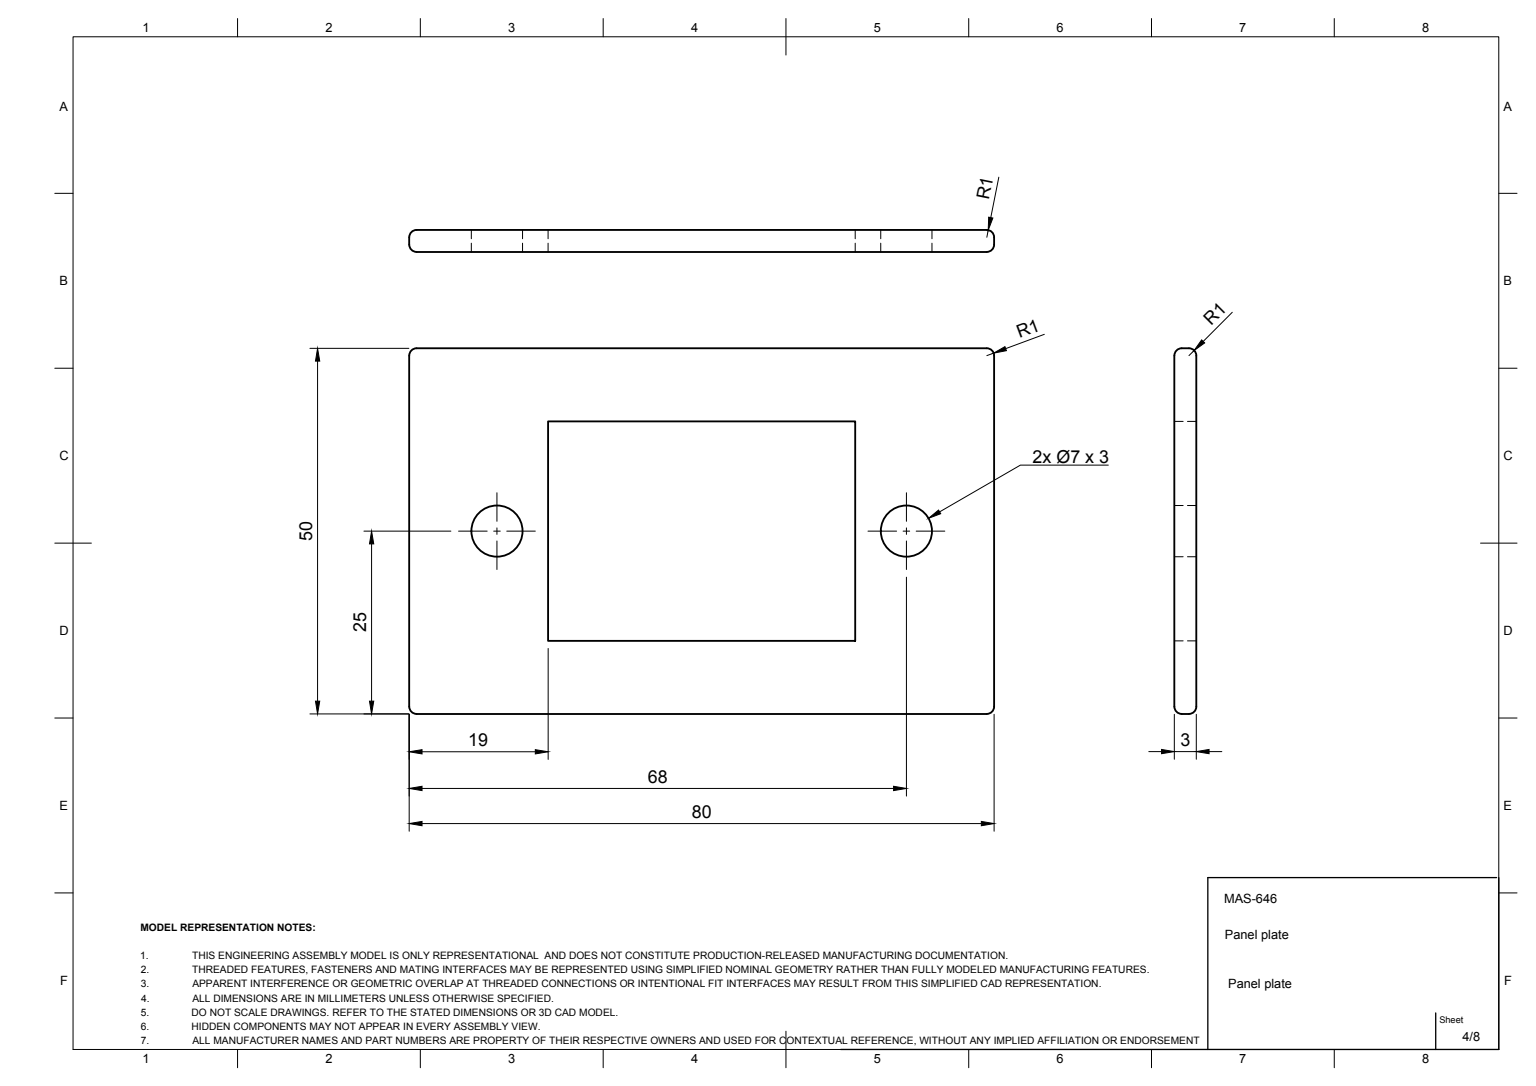
ISO-10303-21;
HEADER;
/* Generated by software containing ST-Developer
 * from STEP Tools, Inc. (www.steptools.com) 
 */

FILE_DESCRIPTION(
/* description */ ('Independent keyed three-contact power inlet for the IEC-connector des
ign category. Longer ground blade, retained contacts, wire termination
 holes and sealed bolted panel interface. Nominal custom interface; IE
C dimensional compatibility and electrical ratings are not assigned.'),

/* implementation_level */ '2;1');

FILE_NAME(
/* name */ 'Panel plate.step',
/* time_stamp */ '2026-11-08T19:55:04-08:00',
/* author */ (''),
/* organization */ (''),
/* preprocessor_version */ 'ST-DEVELOPER v20.2',
/* originating_system */ 'Autodesk Translation Framework v15.17.0.0',
/* authorisation */ '');

FILE_SCHEMA (('AUTOMOTIVE_DESIGN { 1 0 10303 214 3 1 1 }'));
ENDSEC;

DATA;
#10=MECHANICAL_DESIGN_GEOMETRIC_PRESENTATION_REPRESENTATION('',(#110),#21880);
#81=SPHERICAL_SURFACE('',#6694,0.999999999999996);
#82=SPHERICAL_SURFACE('',#6698,0.999999999999996);
#83=SPHERICAL_SURFACE('',#6702,1.);
#84=SPHERICAL_SURFACE('',#6706,0.999999999999996);
#85=SPHERICAL_SURFACE('',#6710,1.);
#86=SPHERICAL_SURFACE('',#6714,0.999999999999996);
#87=SPHERICAL_SURFACE('',#6718,1.);
#88=SPHERICAL_SURFACE('',#6722,1.);
#90=SHAPE_REPRESENTATION_RELATIONSHIP('SRR','None',#21926,#100);
#100=ADVANCED_BREP_SHAPE_REPRESENTATION('',(#120),#21871);
#110=STYLED_ITEM('',(#21985),#120);
#120=MANIFOLD_SOLID_BREP('Body1',#6382);
#159=FACE_BOUND('',#863,.T.);
#160=FACE_BOUND('',#864,.T.);
#161=FACE_BOUND('',#865,.T.);
#162=FACE_BOUND('',#869,.T.);
#163=FACE_BOUND('',#870,.T.);
#164=FACE_BOUND('',#871,.T.);
#233=PLANE('',#6738);
#234=PLANE('',#6739);
#235=PLANE('',#6742);
#236=PLANE('',#6743);
#237=PLANE('',#6744);
#238=PLANE('',#6747);
#239=PLANE('',#6750);
#240=PLANE('',#6751);
#241=PLANE('',#6752);
#242=PLANE('',#6753);
#481=FACE_OUTER_BOUND('',#841,.T.);
#482=FACE_OUTER_BOUND('',#842,.T.);
#483=FACE_OUTER_BOUND('',#843,.T.);
#484=FACE_OUTER_BOUND('',#844,.T.);
#485=FACE_OUTER_BOUND('',#845,.T.);
#486=FACE_OUTER_BOUND('',#846,.T.);
#487=FACE_OUTER_BOUND('',#847,.T.);
#488=FACE_OUTER_BOUND('',#848,.T.);
#489=FACE_OUTER_BOUND('',#849,.T.);
#490=FACE_OUTER_BOUND('',#850,.T.);
#491=FACE_OUTER_BOUND('',#851,.T.);
#492=FACE_OUTER_BOUND('',#852,.T.);
#493=FACE_OUTER_BOUND('',#853,.T.);
#494=FACE_OUTER_BOUND('',#854,.T.);
#495=FACE_OUTER_BOUND('',#855,.T.);
#496=FACE_OUTER_BOUND('',#856,.T.);
#497=FACE_OUTER_BOUND('',#857,.T.);
#498=FACE_OUTER_BOUND('',#858,.T.);
#499=FACE_OUTER_BOUND('',#859,.T.);
#500=FACE_OUTER_BOUND('',#860,.T.);
#501=FACE_OUTER_BOUND('',#861,.T.);
#502=FACE_OUTER_BOUND('',#862,.T.);
#503=FACE_OUTER_BOUND('',#866,.T.);
#504=FACE_OUTER_BOUND('',#867,.T.);
#505=FACE_OUTER_BOUND('',#868,.T.);
#506=FACE_OUTER_BOUND('',#872,.T.);
#507=FACE_OUTER_BOUND('',#873,.T.);
#508=FACE_OUTER_BOUND('',#874,.T.);
#509=FACE_OUTER_BOUND('',#875,.T.);
#510=FACE_OUTER_BOUND('',#876,.T.);
#511=FACE_OUTER_BOUND('',#877,.T.);
#512=FACE_OUTER_BOUND('',#878,.T.);
#841=EDGE_LOOP('',(#4883,#4884,#4885));
#842=EDGE_LOOP('',(#4886,#4887,#4888));
#843=EDGE_LOOP('',(#4889,#4890,#4891));
#844=EDGE_LOOP('',(#4892,#4893,#4894));
#845=EDGE_LOOP('',(#4895,#4896,#4897));
#846=EDGE_LOOP('',(#4898,#4899,#4900));
#847=EDGE_LOOP('',(#4901,#4902,#4903));
#848=EDGE_LOOP('',(#4904,#4905,#4906));
#849=EDGE_LOOP('',(#4907,#4908,#4909,#4910));
#850=EDGE_LOOP('',(#4911,#4912,#4913,#4914));
#851=EDGE_LOOP('',(#4915,#4916,#4917,#4918));
#852=EDGE_LOOP('',(#4919,#4920,#4921,#4922));
#853=EDGE_LOOP('',(#4923,#4924,#4925,#4926));
#854=EDGE_LOOP('',(#4927,#4928,#4929,#4930));
#855=EDGE_LOOP('',(#4931,#4932,#4933,#4934));
#856=EDGE_LOOP('',(#4935,#4936,#4937,#4938));
#857=EDGE_LOOP('',(#4939,#4940,#4941,#4942));
#858=EDGE_LOOP('',(#4943,#4944,#4945,#4946));
#859=EDGE_LOOP('',(#4947,#4948,#4949,#4950));
#860=EDGE_LOOP('',(#4951,#4952,#4953,#4954));
#861=EDGE_LOOP('',(#4955,#4956,#4957,#4958));
#862=EDGE_LOOP('',(#4959,#4960,#4961,#4962));
#863=EDGE_LOOP('',(#4963,#4964,#4965,#4966));
#864=EDGE_LOOP('',(#4967));
#865=EDGE_LOOP('',(#4968));
#866=EDGE_LOOP('',(#4969,#4970,#4971,#4972));
#867=EDGE_LOOP('',(#4973,#4974,#4975,#4976));
#868=EDGE_LOOP('',(#4977,#4978,#4979,#4980));
#869=EDGE_LOOP('',(#4981,#4982,#4983,#4984));
#870=EDGE_LOOP('',(#4985));
#871=EDGE_LOOP('',(#4986));
#872=EDGE_LOOP('',(#4987,#4988,#4989,#4990));
#873=EDGE_LOOP('',(#4991,#4992,#4993,#4994));
#874=EDGE_LOOP('',(#4995,#4996,#4997,#4998));
#875=EDGE_LOOP('',(#4999,#5000,#5001,#5002));
#876=EDGE_LOOP('',(#5003,#5004,#5005,#5006));
#877=EDGE_LOOP('',(#5007,#5008,#5009,#5010));
#878=EDGE_LOOP('',(#5011,#5012,#5013,#5014));
#1096=CIRCLE('',#6695,1.);
#1097=CIRCLE('',#6696,0.999999999999996);
#1098=CIRCLE('',#6697,1.);
#1099=CIRCLE('',#6699,1.);
#1100=CIRCLE('',#6700,0.999999999999996);
#1101=CIRCLE('',#6701,1.);
#1102=CIRCLE('',#6703,0.999999999999996);
#1103=CIRCLE('',#6704,1.);
#1104=CIRCLE('',#6705,1.);
#1105=CIRCLE('',#6707,1.);
#1106=CIRCLE('',#6708,0.999999999999996);
#1107=CIRCLE('',#6709,1.);
#1108=CIRCLE('',#6711,1.);
#1109=CIRCLE('',#6712,1.);
#1110=CIRCLE('',#6713,0.999999999999996);
#1111=CIRCLE('',#6715,1.);
#1112=CIRCLE('',#6716,0.999999999999996);
#1113=CIRCLE('',#6717,1.);
#1114=CIRCLE('',#6719,0.999999999999996);
#1115=CIRCLE('',#6720,1.);
#1116=CIRCLE('',#6721,1.);
#1117=CIRCLE('',#6723,0.999999999999996);
#1118=CIRCLE('',#6724,1.);
#1119=CIRCLE('',#6725,1.);
#1120=CIRCLE('',#6740,3.5);
#1121=CIRCLE('',#6741,3.5);
#1122=CIRCLE('',#6745,3.5);
#1123=CIRCLE('',#6746,3.5);
#1723=LINE('',#16018,#2179);
#1724=LINE('',#16019,#2180);
#1725=LINE('',#16021,#2181);
#1726=LINE('',#16022,#2182);
#1727=LINE('',#16024,#2183);
#1728=LINE('',#16025,#2184);
#1729=LINE('',#16027,#2185);
#1730=LINE('',#16028,#2186);
#1731=LINE('',#16030,#2187);
#1732=LINE('',#16031,#2188);
#1733=LINE('',#16033,#2189);
#1734=LINE('',#16034,#2190);
#1735=LINE('',#16036,#2191);
#1736=LINE('',#16037,#2192);
#1737=LINE('',#16039,#2193);
#1738=LINE('',#16040,#2194);
#1739=LINE('',#16042,#2195);
#1740=LINE('',#16043,#2196);
#1741=LINE('',#16045,#2197);
#1742=LINE('',#16046,#2198);
#1743=LINE('',#16048,#2199);
#1744=LINE('',#16049,#2200);
#1745=LINE('',#16051,#2201);
#1746=LINE('',#16052,#2202);
#1747=LINE('',#16057,#2203);
#1748=LINE('',#16059,#2204);
#1749=LINE('',#16061,#2205);
#1750=LINE('',#16062,#2206);
#1751=LINE('',#16072,#2207);
#1752=LINE('',#16074,#2208);
#1753=LINE('',#16076,#2209);
#1754=LINE('',#16077,#2210);
#1755=LINE('',#16084,#2211);
#1756=LINE('',#16086,#2212);
#1757=LINE('',#16088,#2213);
#1758=LINE('',#16089,#2214);
#1759=LINE('',#16091,#2215);
#1760=LINE('',#16093,#2216);
#2179=VECTOR('',#7611,10.);
#2180=VECTOR('',#7612,10.);
#2181=VECTOR('',#7615,10.);
#2182=VECTOR('',#7616,10.);
#2183=VECTOR('',#7619,10.);
#2184=VECTOR('',#7620,10.);
#2185=VECTOR('',#7623,10.);
#2186=VECTOR('',#7624,10.);
#2187=VECTOR('',#7627,10.);
#2188=VECTOR('',#7628,10.);
#2189=VECTOR('',#7631,10.);
#2190=VECTOR('',#7632,10.);
#2191=VECTOR('',#7635,10.);
#2192=VECTOR('',#7636,10.);
#2193=VECTOR('',#7639,10.);
#2194=VECTOR('',#7640,10.);
#2195=VECTOR('',#7643,10.);
#2196=VECTOR('',#7644,10.);
#2197=VECTOR('',#7647,10.);
#2198=VECTOR('',#7648,10.);
#2199=VECTOR('',#7651,10.);
#2200=VECTOR('',#7652,10.);
#2201=VECTOR('',#7655,10.);
#2202=VECTOR('',#7656,10.);
#2203=VECTOR('',#7661,10.);
#2204=VECTOR('',#7662,10.);
#2205=VECTOR('',#7663,10.);
#2206=VECTOR('',#7664,10.);
#2207=VECTOR('',#7675,10.);
#2208=VECTOR('',#7676,10.);
#2209=VECTOR('',#7677,10.);
#2210=VECTOR('',#7678,10.);
#2211=VECTOR('',#7687,3.5);
#2212=VECTOR('',#7690,3.5);
#2213=VECTOR('',#7693,10.);
#2214=VECTOR('',#7694,10.);
#2215=VECTOR('',#7697,10.);
#2216=VECTOR('',#7700,10.);
#2739=VERTEX_POINT('',#15962);
#2740=VERTEX_POINT('',#15963);
#2741=VERTEX_POINT('',#15965);
#2742=VERTEX_POINT('',#15969);
#2743=VERTEX_POINT('',#15970);
#2744=VERTEX_POINT('',#15972);
#2745=VERTEX_POINT('',#15976);
#2746=VERTEX_POINT('',#15977);
#2747=VERTEX_POINT('',#15979);
#2748=VERTEX_POINT('',#15983);
#2749=VERTEX_POINT('',#15984);
#2750=VERTEX_POINT('',#15986);
#2751=VERTEX_POINT('',#15990);
#2752=VERTEX_POINT('',#15991);
#2753=VERTEX_POINT('',#15993);
#2754=VERTEX_POINT('',#15997);
#2755=VERTEX_POINT('',#15998);
#2756=VERTEX_POINT('',#16000);
#2757=VERTEX_POINT('',#16004);
#2758=VERTEX_POINT('',#16005);
#2759=VERTEX_POINT('',#16007);
#2760=VERTEX_POINT('',#16011);
#2761=VERTEX_POINT('',#16012);
#2762=VERTEX_POINT('',#16014);
#2763=VERTEX_POINT('',#16055);
#2764=VERTEX_POINT('',#16056);
#2765=VERTEX_POINT('',#16058);
#2766=VERTEX_POINT('',#16060);
#2767=VERTEX_POINT('',#16063);
#2768=VERTEX_POINT('',#16065);
#2769=VERTEX_POINT('',#16070);
#2770=VERTEX_POINT('',#16071);
#2771=VERTEX_POINT('',#16073);
#2772=VERTEX_POINT('',#16075);
#2773=VERTEX_POINT('',#16078);
#2774=VERTEX_POINT('',#16080);
#3501=EDGE_CURVE('',#2739,#2740,#1096,.F.);
#3502=EDGE_CURVE('',#2741,#2739,#1097,.F.);
#3503=EDGE_CURVE('',#2740,#2741,#1098,.F.);
#3504=EDGE_CURVE('',#2742,#2743,#1099,.F.);
#3505=EDGE_CURVE('',#2744,#2742,#1100,.F.);
#3506=EDGE_CURVE('',#2743,#2744,#1101,.F.);
#3507=EDGE_CURVE('',#2745,#2746,#1102,.F.);
#3508=EDGE_CURVE('',#2747,#2745,#1103,.F.);
#3509=EDGE_CURVE('',#2746,#2747,#1104,.F.);
#3510=EDGE_CURVE('',#2748,#2749,#1105,.F.);
#3511=EDGE_CURVE('',#2750,#2748,#1106,.F.);
#3512=EDGE_CURVE('',#2749,#2750,#1107,.F.);
#3513=EDGE_CURVE('',#2751,#2752,#1108,.F.);
#3514=EDGE_CURVE('',#2753,#2751,#1109,.F.);
#3515=EDGE_CURVE('',#2752,#2753,#1110,.F.);
#3516=EDGE_CURVE('',#2754,#2755,#1111,.F.);
#3517=EDGE_CURVE('',#2756,#2754,#1112,.F.);
#3518=EDGE_CURVE('',#2755,#2756,#1113,.F.);
#3519=EDGE_CURVE('',#2757,#2758,#1114,.F.);
#3520=EDGE_CURVE('',#2759,#2757,#1115,.F.);
#3521=EDGE_CURVE('',#2758,#2759,#1116,.F.);
#3522=EDGE_CURVE('',#2760,#2761,#1117,.F.);
#3523=EDGE_CURVE('',#2762,#2760,#1118,.F.);
#3524=EDGE_CURVE('',#2761,#2762,#1119,.F.);
#3525=EDGE_CURVE('',#2760,#2753,#1723,.T.);
#3526=EDGE_CURVE('',#2751,#2762,#1724,.T.);
#3527=EDGE_CURVE('',#2757,#2761,#1725,.T.);
#3528=EDGE_CURVE('',#2762,#2759,#1726,.T.);
#3529=EDGE_CURVE('',#2754,#2760,#1727,.T.);
#3530=EDGE_CURVE('',#2761,#2756,#1728,.T.);
#3531=EDGE_CURVE('',#2745,#2758,#1729,.T.);
#3532=EDGE_CURVE('',#2759,#2747,#1730,.T.);
#3533=EDGE_CURVE('',#2748,#2757,#1731,.T.);
#3534=EDGE_CURVE('',#2758,#2750,#1732,.T.);
#3535=EDGE_CURVE('',#2749,#2755,#1733,.T.);
#3536=EDGE_CURVE('',#2756,#2748,#1734,.T.);
#3537=EDGE_CURVE('',#2755,#2743,#1735,.T.);
#3538=EDGE_CURVE('',#2744,#2754,#1736,.T.);
#3539=EDGE_CURVE('',#2742,#2752,#1737,.T.);
#3540=EDGE_CURVE('',#2753,#2744,#1738,.T.);
#3541=EDGE_CURVE('',#2752,#2746,#1739,.T.);
#3542=EDGE_CURVE('',#2747,#2751,#1740,.T.);
#3543=EDGE_CURVE('',#2740,#2749,#1741,.T.);
#3544=EDGE_CURVE('',#2750,#2739,#1742,.T.);
#3545=EDGE_CURVE('',#2739,#2745,#1743,.T.);
#3546=EDGE_CURVE('',#2746,#2741,#1744,.T.);
#3547=EDGE_CURVE('',#2743,#2740,#1745,.T.);
#3548=EDGE_CURVE('',#2741,#2742,#1746,.T.);
#3549=EDGE_CURVE('',#2763,#2764,#1747,.T.);
#3550=EDGE_CURVE('',#2764,#2765,#1748,.T.);
#3551=EDGE_CURVE('',#2765,#2766,#1749,.T.);
#3552=EDGE_CURVE('',#2766,#2763,#1750,.T.);
#3553=EDGE_CURVE('',#2767,#2767,#1120,.T.);
#3554=EDGE_CURVE('',#2768,#2768,#1121,.T.);
#3555=EDGE_CURVE('',#2769,#2770,#1751,.T.);
#3556=EDGE_CURVE('',#2770,#2771,#1752,.T.);
#3557=EDGE_CURVE('',#2771,#2772,#1753,.T.);
#3558=EDGE_CURVE('',#2772,#2769,#1754,.T.);
#3559=EDGE_CURVE('',#2773,#2773,#1122,.T.);
#3560=EDGE_CURVE('',#2774,#2774,#1123,.T.);
#3561=EDGE_CURVE('',#2774,#2768,#1755,.T.);
#3562=EDGE_CURVE('',#2773,#2767,#1756,.T.);
#3563=EDGE_CURVE('',#2769,#2764,#1757,.T.);
#3564=EDGE_CURVE('',#2770,#2763,#1758,.T.);
#3565=EDGE_CURVE('',#2772,#2765,#1759,.T.);
#3566=EDGE_CURVE('',#2771,#2766,#1760,.T.);
#4883=ORIENTED_EDGE('',*,*,#3501,.F.);
#4884=ORIENTED_EDGE('',*,*,#3502,.F.);
#4885=ORIENTED_EDGE('',*,*,#3503,.F.);
#4886=ORIENTED_EDGE('',*,*,#3504,.F.);
#4887=ORIENTED_EDGE('',*,*,#3505,.F.);
#4888=ORIENTED_EDGE('',*,*,#3506,.F.);
#4889=ORIENTED_EDGE('',*,*,#3507,.F.);
#4890=ORIENTED_EDGE('',*,*,#3508,.F.);
#4891=ORIENTED_EDGE('',*,*,#3509,.F.);
#4892=ORIENTED_EDGE('',*,*,#3510,.F.);
#4893=ORIENTED_EDGE('',*,*,#3511,.F.);
#4894=ORIENTED_EDGE('',*,*,#3512,.F.);
#4895=ORIENTED_EDGE('',*,*,#3513,.F.);
#4896=ORIENTED_EDGE('',*,*,#3514,.F.);
#4897=ORIENTED_EDGE('',*,*,#3515,.F.);
#4898=ORIENTED_EDGE('',*,*,#3516,.F.);
#4899=ORIENTED_EDGE('',*,*,#3517,.F.);
#4900=ORIENTED_EDGE('',*,*,#3518,.F.);
#4901=ORIENTED_EDGE('',*,*,#3519,.F.);
#4902=ORIENTED_EDGE('',*,*,#3520,.F.);
#4903=ORIENTED_EDGE('',*,*,#3521,.F.);
#4904=ORIENTED_EDGE('',*,*,#3522,.F.);
#4905=ORIENTED_EDGE('',*,*,#3523,.F.);
#4906=ORIENTED_EDGE('',*,*,#3524,.F.);
#4907=ORIENTED_EDGE('',*,*,#3523,.T.);
#4908=ORIENTED_EDGE('',*,*,#3525,.T.);
#4909=ORIENTED_EDGE('',*,*,#3514,.T.);
#4910=ORIENTED_EDGE('',*,*,#3526,.T.);
#4911=ORIENTED_EDGE('',*,*,#3520,.T.);
#4912=ORIENTED_EDGE('',*,*,#3527,.T.);
#4913=ORIENTED_EDGE('',*,*,#3524,.T.);
#4914=ORIENTED_EDGE('',*,*,#3528,.T.);
#4915=ORIENTED_EDGE('',*,*,#3517,.T.);
#4916=ORIENTED_EDGE('',*,*,#3529,.T.);
#4917=ORIENTED_EDGE('',*,*,#3522,.T.);
#4918=ORIENTED_EDGE('',*,*,#3530,.T.);
#4919=ORIENTED_EDGE('',*,*,#3508,.T.);
#4920=ORIENTED_EDGE('',*,*,#3531,.T.);
#4921=ORIENTED_EDGE('',*,*,#3521,.T.);
#4922=ORIENTED_EDGE('',*,*,#3532,.T.);
#4923=ORIENTED_EDGE('',*,*,#3511,.T.);
#4924=ORIENTED_EDGE('',*,*,#3533,.T.);
#4925=ORIENTED_EDGE('',*,*,#3519,.T.);
#4926=ORIENTED_EDGE('',*,*,#3534,.T.);
#4927=ORIENTED_EDGE('',*,*,#3510,.T.);
#4928=ORIENTED_EDGE('',*,*,#3535,.T.);
#4929=ORIENTED_EDGE('',*,*,#3518,.T.);
#4930=ORIENTED_EDGE('',*,*,#3536,.T.);
#4931=ORIENTED_EDGE('',*,*,#3516,.T.);
#4932=ORIENTED_EDGE('',*,*,#3537,.T.);
#4933=ORIENTED_EDGE('',*,*,#3506,.T.);
#4934=ORIENTED_EDGE('',*,*,#3538,.T.);
#4935=ORIENTED_EDGE('',*,*,#3505,.T.);
#4936=ORIENTED_EDGE('',*,*,#3539,.T.);
#4937=ORIENTED_EDGE('',*,*,#3515,.T.);
#4938=ORIENTED_EDGE('',*,*,#3540,.T.);
#4939=ORIENTED_EDGE('',*,*,#3513,.T.);
#4940=ORIENTED_EDGE('',*,*,#3541,.T.);
#4941=ORIENTED_EDGE('',*,*,#3509,.T.);
#4942=ORIENTED_EDGE('',*,*,#3542,.T.);
#4943=ORIENTED_EDGE('',*,*,#3501,.T.);
#4944=ORIENTED_EDGE('',*,*,#3543,.T.);
#4945=ORIENTED_EDGE('',*,*,#3512,.T.);
#4946=ORIENTED_EDGE('',*,*,#3544,.T.);
#4947=ORIENTED_EDGE('',*,*,#3502,.T.);
#4948=ORIENTED_EDGE('',*,*,#3545,.T.);
#4949=ORIENTED_EDGE('',*,*,#3507,.T.);
#4950=ORIENTED_EDGE('',*,*,#3546,.T.);
#4951=ORIENTED_EDGE('',*,*,#3504,.T.);
#4952=ORIENTED_EDGE('',*,*,#3547,.T.);
#4953=ORIENTED_EDGE('',*,*,#3503,.T.);
#4954=ORIENTED_EDGE('',*,*,#3548,.T.);
#4955=ORIENTED_EDGE('',*,*,#3525,.F.);
#4956=ORIENTED_EDGE('',*,*,#3529,.F.);
#4957=ORIENTED_EDGE('',*,*,#3538,.F.);
#4958=ORIENTED_EDGE('',*,*,#3540,.F.);
#4959=ORIENTED_EDGE('',*,*,#3526,.F.);
#4960=ORIENTED_EDGE('',*,*,#3542,.F.);
#4961=ORIENTED_EDGE('',*,*,#3532,.F.);
#4962=ORIENTED_EDGE('',*,*,#3528,.F.);
#4963=ORIENTED_EDGE('',*,*,#3549,.T.);
#4964=ORIENTED_EDGE('',*,*,#3550,.T.);
#4965=ORIENTED_EDGE('',*,*,#3551,.T.);
#4966=ORIENTED_EDGE('',*,*,#3552,.T.);
#4967=ORIENTED_EDGE('',*,*,#3553,.T.);
#4968=ORIENTED_EDGE('',*,*,#3554,.T.);
#4969=ORIENTED_EDGE('',*,*,#3527,.F.);
#4970=ORIENTED_EDGE('',*,*,#3533,.F.);
#4971=ORIENTED_EDGE('',*,*,#3536,.F.);
#4972=ORIENTED_EDGE('',*,*,#3530,.F.);
#4973=ORIENTED_EDGE('',*,*,#3531,.F.);
#4974=ORIENTED_EDGE('',*,*,#3545,.F.);
#4975=ORIENTED_EDGE('',*,*,#3544,.F.);
#4976=ORIENTED_EDGE('',*,*,#3534,.F.);
#4977=ORIENTED_EDGE('',*,*,#3535,.F.);
#4978=ORIENTED_EDGE('',*,*,#3543,.F.);
#4979=ORIENTED_EDGE('',*,*,#3547,.F.);
#4980=ORIENTED_EDGE('',*,*,#3537,.F.);
#4981=ORIENTED_EDGE('',*,*,#3555,.T.);
#4982=ORIENTED_EDGE('',*,*,#3556,.T.);
#4983=ORIENTED_EDGE('',*,*,#3557,.T.);
#4984=ORIENTED_EDGE('',*,*,#3558,.T.);
#4985=ORIENTED_EDGE('',*,*,#3559,.T.);
#4986=ORIENTED_EDGE('',*,*,#3560,.T.);
#4987=ORIENTED_EDGE('',*,*,#3539,.F.);
#4988=ORIENTED_EDGE('',*,*,#3548,.F.);
#4989=ORIENTED_EDGE('',*,*,#3546,.F.);
#4990=ORIENTED_EDGE('',*,*,#3541,.F.);
#4991=ORIENTED_EDGE('',*,*,#3560,.F.);
#4992=ORIENTED_EDGE('',*,*,#3561,.T.);
#4993=ORIENTED_EDGE('',*,*,#3554,.F.);
#4994=ORIENTED_EDGE('',*,*,#3561,.F.);
#4995=ORIENTED_EDGE('',*,*,#3559,.F.);
#4996=ORIENTED_EDGE('',*,*,#3562,.T.);
#4997=ORIENTED_EDGE('',*,*,#3553,.F.);
#4998=ORIENTED_EDGE('',*,*,#3562,.F.);
#4999=ORIENTED_EDGE('',*,*,#3555,.F.);
#5000=ORIENTED_EDGE('',*,*,#3563,.T.);
#5001=ORIENTED_EDGE('',*,*,#3549,.F.);
#5002=ORIENTED_EDGE('',*,*,#3564,.F.);
#5003=ORIENTED_EDGE('',*,*,#3558,.F.);
#5004=ORIENTED_EDGE('',*,*,#3565,.T.);
#5005=ORIENTED_EDGE('',*,*,#3550,.F.);
#5006=ORIENTED_EDGE('',*,*,#3563,.F.);
#5007=ORIENTED_EDGE('',*,*,#3557,.F.);
#5008=ORIENTED_EDGE('',*,*,#3566,.T.);
#5009=ORIENTED_EDGE('',*,*,#3551,.F.);
#5010=ORIENTED_EDGE('',*,*,#3565,.F.);
#5011=ORIENTED_EDGE('',*,*,#3556,.F.);
#5012=ORIENTED_EDGE('',*,*,#3564,.T.);
#5013=ORIENTED_EDGE('',*,*,#3552,.F.);
#5014=ORIENTED_EDGE('',*,*,#3566,.F.);
#5943=CYLINDRICAL_SURFACE('',#6726,1.);
#5944=CYLINDRICAL_SURFACE('',#6727,1.);
#5945=CYLINDRICAL_SURFACE('',#6728,1.);
#5946=CYLINDRICAL_SURFACE('',#6729,1.);
#5947=CYLINDRICAL_SURFACE('',#6730,1.);
#5948=CYLINDRICAL_SURFACE('',#6731,1.);
#5949=CYLINDRICAL_SURFACE('',#6732,1.);
#5950=CYLINDRICAL_SURFACE('',#6733,1.);
#5951=CYLINDRICAL_SURFACE('',#6734,1.);
#5952=CYLINDRICAL_SURFACE('',#6735,1.);
#5953=CYLINDRICAL_SURFACE('',#6736,1.);
#5954=CYLINDRICAL_SURFACE('',#6737,1.);
#5955=CYLINDRICAL_SURFACE('',#6748,3.5);
#5956=CYLINDRICAL_SURFACE('',#6749,3.5);
#6193=ADVANCED_FACE('',(#481),#81,.T.);
#6194=ADVANCED_FACE('',(#482),#82,.T.);
#6195=ADVANCED_FACE('',(#483),#83,.T.);
#6196=ADVANCED_FACE('',(#484),#84,.T.);
#6197=ADVANCED_FACE('',(#485),#85,.T.);
#6198=ADVANCED_FACE('',(#486),#86,.T.);
#6199=ADVANCED_FACE('',(#487),#87,.T.);
#6200=ADVANCED_FACE('',(#488),#88,.T.);
#6201=ADVANCED_FACE('',(#489),#5943,.T.);
#6202=ADVANCED_FACE('',(#490),#5944,.T.);
#6203=ADVANCED_FACE('',(#491),#5945,.T.);
#6204=ADVANCED_FACE('',(#492),#5946,.T.);
#6205=ADVANCED_FACE('',(#493),#5947,.T.);
#6206=ADVANCED_FACE('',(#494),#5948,.T.);
#6207=ADVANCED_FACE('',(#495),#5949,.T.);
#6208=ADVANCED_FACE('',(#496),#5950,.T.);
#6209=ADVANCED_FACE('',(#497),#5951,.T.);
#6210=ADVANCED_FACE('',(#498),#5952,.T.);
#6211=ADVANCED_FACE('',(#499),#5953,.T.);
#6212=ADVANCED_FACE('',(#500),#5954,.T.);
#6213=ADVANCED_FACE('',(#501),#233,.T.);
#6214=ADVANCED_FACE('',(#502,#159,#160,#161),#234,.F.);
#6215=ADVANCED_FACE('',(#503),#235,.T.);
#6216=ADVANCED_FACE('',(#504),#236,.T.);
#6217=ADVANCED_FACE('',(#505,#162,#163,#164),#237,.T.);
#6218=ADVANCED_FACE('',(#506),#238,.T.);
#6219=ADVANCED_FACE('',(#507),#5955,.F.);
#6220=ADVANCED_FACE('',(#508),#5956,.F.);
#6221=ADVANCED_FACE('',(#509),#239,.F.);
#6222=ADVANCED_FACE('',(#510),#240,.F.);
#6223=ADVANCED_FACE('',(#511),#241,.F.);
#6224=ADVANCED_FACE('',(#512),#242,.F.);
#6382=CLOSED_SHELL('',(#6193,#6194,#6195,#6196,#6197,#6198,#6199,#6200,
#6201,#6202,#6203,#6204,#6205,#6206,#6207,#6208,#6209,#6210,#6211,#6212,
#6213,#6214,#6215,#6216,#6217,#6218,#6219,#6220,#6221,#6222,#6223,#6224));
#6693=AXIS2_PLACEMENT_3D('',#15960,#7543,#7544);
#6694=AXIS2_PLACEMENT_3D('',#15961,#7545,#7546);
#6695=AXIS2_PLACEMENT_3D('',#15964,#7547,#7548);
#6696=AXIS2_PLACEMENT_3D('',#15966,#7549,#7550);
#6697=AXIS2_PLACEMENT_3D('',#15967,#7551,#7552);
#6698=AXIS2_PLACEMENT_3D('',#15968,#7553,#7554);
#6699=AXIS2_PLACEMENT_3D('',#15971,#7555,#7556);
#6700=AXIS2_PLACEMENT_3D('',#15973,#7557,#7558);
#6701=AXIS2_PLACEMENT_3D('',#15974,#7559,#7560);
#6702=AXIS2_PLACEMENT_3D('',#15975,#7561,#7562);
#6703=AXIS2_PLACEMENT_3D('',#15978,#7563,#7564);
#6704=AXIS2_PLACEMENT_3D('',#15980,#7565,#7566);
#6705=AXIS2_PLACEMENT_3D('',#15981,#7567,#7568);
#6706=AXIS2_PLACEMENT_3D('',#15982,#7569,#7570);
#6707=AXIS2_PLACEMENT_3D('',#15985,#7571,#7572);
#6708=AXIS2_PLACEMENT_3D('',#15987,#7573,#7574);
#6709=AXIS2_PLACEMENT_3D('',#15988,#7575,#7576);
#6710=AXIS2_PLACEMENT_3D('',#15989,#7577,#7578);
#6711=AXIS2_PLACEMENT_3D('',#15992,#7579,#7580);
#6712=AXIS2_PLACEMENT_3D('',#15994,#7581,#7582);
#6713=AXIS2_PLACEMENT_3D('',#15995,#7583,#7584);
#6714=AXIS2_PLACEMENT_3D('',#15996,#7585,#7586);
#6715=AXIS2_PLACEMENT_3D('',#15999,#7587,#7588);
#6716=AXIS2_PLACEMENT_3D('',#16001,#7589,#7590);
#6717=AXIS2_PLACEMENT_3D('',#16002,#7591,#7592);
#6718=AXIS2_PLACEMENT_3D('',#16003,#7593,#7594);
#6719=AXIS2_PLACEMENT_3D('',#16006,#7595,#7596);
#6720=AXIS2_PLACEMENT_3D('',#16008,#7597,#7598);
#6721=AXIS2_PLACEMENT_3D('',#16009,#7599,#7600);
#6722=AXIS2_PLACEMENT_3D('',#16010,#7601,#7602);
#6723=AXIS2_PLACEMENT_3D('',#16013,#7603,#7604);
#6724=AXIS2_PLACEMENT_3D('',#16015,#7605,#7606);
#6725=AXIS2_PLACEMENT_3D('',#16016,#7607,#7608);
#6726=AXIS2_PLACEMENT_3D('',#16017,#7609,#7610);
#6727=AXIS2_PLACEMENT_3D('',#16020,#7613,#7614);
#6728=AXIS2_PLACEMENT_3D('',#16023,#7617,#7618);
#6729=AXIS2_PLACEMENT_3D('',#16026,#7621,#7622);
#6730=AXIS2_PLACEMENT_3D('',#16029,#7625,#7626);
#6731=AXIS2_PLACEMENT_3D('',#16032,#7629,#7630);
#6732=AXIS2_PLACEMENT_3D('',#16035,#7633,#7634);
#6733=AXIS2_PLACEMENT_3D('',#16038,#7637,#7638);
#6734=AXIS2_PLACEMENT_3D('',#16041,#7641,#7642);
#6735=AXIS2_PLACEMENT_3D('',#16044,#7645,#7646);
#6736=AXIS2_PLACEMENT_3D('',#16047,#7649,#7650);
#6737=AXIS2_PLACEMENT_3D('',#16050,#7653,#7654);
#6738=AXIS2_PLACEMENT_3D('',#16053,#7657,#7658);
#6739=AXIS2_PLACEMENT_3D('',#16054,#7659,#7660);
#6740=AXIS2_PLACEMENT_3D('',#16064,#7665,#7666);
#6741=AXIS2_PLACEMENT_3D('',#16066,#7667,#7668);
#6742=AXIS2_PLACEMENT_3D('',#16067,#7669,#7670);
#6743=AXIS2_PLACEMENT_3D('',#16068,#7671,#7672);
#6744=AXIS2_PLACEMENT_3D('',#16069,#7673,#7674);
#6745=AXIS2_PLACEMENT_3D('',#16079,#7679,#7680);
#6746=AXIS2_PLACEMENT_3D('',#16081,#7681,#7682);
#6747=AXIS2_PLACEMENT_3D('',#16082,#7683,#7684);
#6748=AXIS2_PLACEMENT_3D('',#16083,#7685,#7686);
#6749=AXIS2_PLACEMENT_3D('',#16085,#7688,#7689);
#6750=AXIS2_PLACEMENT_3D('',#16087,#7691,#7692);
#6751=AXIS2_PLACEMENT_3D('',#16090,#7695,#7696);
#6752=AXIS2_PLACEMENT_3D('',#16092,#7698,#7699);
#6753=AXIS2_PLACEMENT_3D('',#16094,#7701,#7702);
#7543=DIRECTION('axis',(0.,0.,1.));
#7544=DIRECTION('refdir',(1.,0.,0.));
#7545=DIRECTION('center_axis',(0.408248290463861,-0.816496580927726,0.408248290463864));
#7546=DIRECTION('ref_axis',(0.577350269189625,0.577350269189625,0.577350269189629));
#7547=DIRECTION('center_axis',(0.,1.,4.44089209850063E-15));
#7548=DIRECTION('ref_axis',(1.,0.,0.));
#7549=DIRECTION('center_axis',(0.,0.,1.));
#7550=DIRECTION('ref_axis',(0.,1.,0.));
#7551=DIRECTION('center_axis',(1.,-4.44089209850062E-15,0.));
#7552=DIRECTION('ref_axis',(0.,0.,1.));
#7553=DIRECTION('center_axis',(-0.40824829046386,-0.816496580927728,0.408248290463862));
#7554=DIRECTION('ref_axis',(-0.577350269189625,0.577350269189625,0.577350269189628));
#7555=DIRECTION('center_axis',(-1.,0.,0.));
#7556=DIRECTION('ref_axis',(0.,1.,0.));
#7557=DIRECTION('center_axis',(0.,0.,1.));
#7558=DIRECTION('ref_axis',(-1.,0.,0.));
#7559=DIRECTION('center_axis',(4.44089209850062E-15,1.,0.));
#7560=DIRECTION('ref_axis',(0.,0.,1.));
#7561=DIRECTION('center_axis',(-0.816496580927725,0.408248290463866,-0.408248290463862));
#7562=DIRECTION('ref_axis',(0.577350269189629,0.577350269189625,-0.577350269189623));
#7563=DIRECTION('center_axis',(0.,0.,-1.));
#7564=DIRECTION('ref_axis',(1.,0.,0.));
#7565=DIRECTION('center_axis',(-4.44089209850062E-15,1.,0.));
#7566=DIRECTION('ref_axis',(0.,0.,-1.));
#7567=DIRECTION('center_axis',(1.,0.,-4.44089209850063E-15));
#7568=DIRECTION('ref_axis',(0.,1.,0.));
#7569=DIRECTION('center_axis',(-0.408248290463861,-0.816496580927728,-0.408248290463861));
#7570=DIRECTION('ref_axis',(0.577350269189625,-0.577350269189625,0.577350269189628));
#7571=DIRECTION('center_axis',(1.,0.,0.));
#7572=DIRECTION('ref_axis',(0.,-1.,0.));
#7573=DIRECTION('center_axis',(0.,0.,1.));
#7574=DIRECTION('ref_axis',(1.,0.,0.));
#7575=DIRECTION('center_axis',(-4.44089209850062E-15,-1.,0.));
#7576=DIRECTION('ref_axis',(0.,0.,1.));
#7577=DIRECTION('center_axis',(0.408248290463867,-0.408248290463859,-0.816496580927726));
#7578=DIRECTION('ref_axis',(-0.577350269189629,0.577350269189622,-0.577350269189626));
#7579=DIRECTION('center_axis',(-1.,0.,0.));
#7580=DIRECTION('ref_axis',(0.,0.,-1.));
#7581=DIRECTION('center_axis',(0.,1.,-4.44089209850063E-15));
#7582=DIRECTION('ref_axis',(-1.,0.,0.));
#7583=DIRECTION('center_axis',(0.,0.,-1.));
#7584=DIRECTION('ref_axis',(0.,1.,0.));
#7585=DIRECTION('center_axis',(0.408248290463861,-0.816496580927726,-0.408248290463864));
#7586=DIRECTION('ref_axis',(-0.577350269189625,-0.577350269189625,0.577350269189629));
#7587=DIRECTION('center_axis',(0.,-1.,4.44089209850063E-15));
#7588=DIRECTION('ref_axis',(-1.,0.,0.));
#7589=DIRECTION('center_axis',(0.,0.,1.));
#7590=DIRECTION('ref_axis',(0.,-1.,0.));
#7591=DIRECTION('center_axis',(-1.,4.44089209850062E-15,0.));
#7592=DIRECTION('ref_axis',(0.,0.,1.));
#7593=DIRECTION('center_axis',(-0.816496580927729,-0.408248290463861,-0.40824829046386));
#7594=DIRECTION('ref_axis',(0.577350269189622,-0.577350269189629,-0.577350269189626));
#7595=DIRECTION('center_axis',(0.,0.,-1.));
#7596=DIRECTION('ref_axis',(0.,-1.,0.));
#7597=DIRECTION('center_axis',(1.,0.,0.));
#7598=DIRECTION('ref_axis',(0.,0.,-1.));
#7599=DIRECTION('center_axis',(0.,-1.,-4.44089209850063E-15));
#7600=DIRECTION('ref_axis',(1.,0.,0.));
#7601=DIRECTION('center_axis',(-0.816496580927726,0.408248290463863,0.408248290463863));
#7602=DIRECTION('ref_axis',(-0.577350269189629,-0.577350269189625,-0.577350269189623));
#7603=DIRECTION('center_axis',(0.,0.,-1.));
#7604=DIRECTION('ref_axis',(-1.,0.,0.));
#7605=DIRECTION('center_axis',(4.44089209850062E-15,-1.,0.));
#7606=DIRECTION('ref_axis',(0.,0.,-1.));
#7607=DIRECTION('center_axis',(-1.,0.,-4.44089209850063E-15));
#7608=DIRECTION('ref_axis',(0.,-1.,0.));
#7609=DIRECTION('center_axis',(0.,-1.,0.));
#7610=DIRECTION('ref_axis',(-0.707106781186549,0.,-0.707106781186546));
#7611=DIRECTION('',(0.,1.,0.));
#7612=DIRECTION('',(0.,-1.,0.));
#7613=DIRECTION('center_axis',(1.,0.,0.));
#7614=DIRECTION('ref_axis',(0.,-0.707106781186549,-0.707106781186546));
#7615=DIRECTION('',(-1.,0.,0.));
#7616=DIRECTION('',(1.,0.,0.));
#7617=DIRECTION('center_axis',(0.,0.,1.));
#7618=DIRECTION('ref_axis',(-0.707106781186548,-0.707106781186548,0.));
#7619=DIRECTION('',(0.,0.,-1.));
#7620=DIRECTION('',(0.,0.,1.));
#7621=DIRECTION('center_axis',(0.,1.,0.));
#7622=DIRECTION('ref_axis',(0.707106781186549,0.,-0.707106781186546));
#7623=DIRECTION('',(0.,-1.,0.));
#7624=DIRECTION('',(0.,1.,0.));
#7625=DIRECTION('center_axis',(0.,0.,1.));
#7626=DIRECTION('ref_axis',(0.707106781186548,-0.707106781186548,0.));
#7627=DIRECTION('',(0.,0.,-1.));
#7628=DIRECTION('',(0.,0.,1.));
#7629=DIRECTION('center_axis',(1.,0.,0.));
#7630=DIRECTION('ref_axis',(0.,-0.707106781186549,0.707106781186546));
#7631=DIRECTION('',(-1.,0.,0.));
#7632=DIRECTION('',(1.,0.,0.));
#7633=DIRECTION('center_axis',(0.,-1.,0.));
#7634=DIRECTION('ref_axis',(-0.707106781186549,0.,0.707106781186546));
#7635=DIRECTION('',(0.,1.,0.));
#7636=DIRECTION('',(0.,-1.,0.));
#7637=DIRECTION('center_axis',(0.,0.,1.));
#7638=DIRECTION('ref_axis',(-0.707106781186548,0.707106781186548,0.));
#7639=DIRECTION('',(0.,0.,-1.));
#7640=DIRECTION('',(0.,0.,1.));
#7641=DIRECTION('center_axis',(-1.,0.,0.));
#7642=DIRECTION('ref_axis',(0.,0.707106781186549,-0.707106781186546));
#7643=DIRECTION('',(1.,0.,0.));
#7644=DIRECTION('',(-1.,0.,0.));
#7645=DIRECTION('center_axis',(0.,1.,0.));
#7646=DIRECTION('ref_axis',(0.707106781186549,0.,0.707106781186546));
#7647=DIRECTION('',(0.,-1.,0.));
#7648=DIRECTION('',(0.,1.,0.));
#7649=DIRECTION('center_axis',(0.,0.,1.));
#7650=DIRECTION('ref_axis',(0.707106781186548,0.707106781186548,0.));
#7651=DIRECTION('',(0.,0.,-1.));
#7652=DIRECTION('',(0.,0.,1.));
#7653=DIRECTION('center_axis',(-1.,0.,0.));
#7654=DIRECTION('ref_axis',(0.,0.707106781186549,0.707106781186546));
#7655=DIRECTION('',(1.,0.,0.));
#7656=DIRECTION('',(-1.,0.,0.));
#7657=DIRECTION('center_axis',(-1.,0.,0.));
#7658=DIRECTION('ref_axis',(0.,-1.,0.));
#7659=DIRECTION('center_axis',(0.,0.,1.));
#7660=DIRECTION('ref_axis',(1.,0.,0.));
#7661=DIRECTION('',(1.,0.,0.));
#7662=DIRECTION('',(0.,1.,0.));
#7663=DIRECTION('',(-1.,0.,0.));
#7664=DIRECTION('',(0.,-1.,0.));
#7665=DIRECTION('center_axis',(0.,0.,1.));
#7666=DIRECTION('ref_axis',(1.,0.,0.));
#7667=DIRECTION('center_axis',(0.,0.,1.));
#7668=DIRECTION('ref_axis',(1.,0.,0.));
#7669=DIRECTION('center_axis',(0.,-1.,0.));
#7670=DIRECTION('ref_axis',(1.,0.,0.));
#7671=DIRECTION('center_axis',(1.,0.,0.));
#7672=DIRECTION('ref_axis',(0.,1.,0.));
#7673=DIRECTION('center_axis',(0.,0.,1.));
#7674=DIRECTION('ref_axis',(1.,0.,0.));
#7675=DIRECTION('',(-1.,0.,0.));
#7676=DIRECTION('',(0.,1.,0.));
#7677=DIRECTION('',(1.,0.,0.));
#7678=DIRECTION('',(0.,-1.,0.));
#7679=DIRECTION('center_axis',(0.,0.,-1.));
#7680=DIRECTION('ref_axis',(1.,0.,0.));
#7681=DIRECTION('center_axis',(0.,0.,-1.));
#7682=DIRECTION('ref_axis',(1.,0.,0.));
#7683=DIRECTION('center_axis',(0.,1.,0.));
#7684=DIRECTION('ref_axis',(-1.,0.,0.));
#7685=DIRECTION('center_axis',(0.,0.,-1.));
#7686=DIRECTION('ref_axis',(1.,0.,0.));
#7687=DIRECTION('',(0.,0.,-1.));
#7688=DIRECTION('center_axis',(0.,0.,-1.));
#7689=DIRECTION('ref_axis',(1.,0.,0.));
#7690=DIRECTION('',(0.,0.,-1.));
#7691=DIRECTION('center_axis',(0.,-1.,0.));
#7692=DIRECTION('ref_axis',(-1.,0.,0.));
#7693=DIRECTION('',(0.,0.,-1.));
#7694=DIRECTION('',(0.,0.,-1.));
#7695=DIRECTION('center_axis',(1.,0.,0.));
#7696=DIRECTION('ref_axis',(0.,-1.,0.));
#7697=DIRECTION('',(0.,0.,-1.));
#7698=DIRECTION('center_axis',(0.,1.,0.));
#7699=DIRECTION('ref_axis',(1.,0.,0.));
#7700=DIRECTION('',(0.,0.,-1.));
#7701=DIRECTION('center_axis',(-1.,0.,0.));
#7702=DIRECTION('ref_axis',(0.,1.,0.));
#15960=CARTESIAN_POINT('',(0.,0.,0.));
#15961=CARTESIAN_POINT('Origin',(39.,24.,2.));
#15962=CARTESIAN_POINT('',(40.,24.,2.));
#15963=CARTESIAN_POINT('',(39.,24.,3.));
#15964=CARTESIAN_POINT('Origin',(39.,24.,2.));
#15965=CARTESIAN_POINT('',(39.,25.,2.));
#15966=CARTESIAN_POINT('Origin',(39.,24.,2.));
#15967=CARTESIAN_POINT('Origin',(39.,24.,2.));
#15968=CARTESIAN_POINT('Origin',(-39.,24.,2.));
#15969=CARTESIAN_POINT('',(-39.,25.,2.));
#15970=CARTESIAN_POINT('',(-39.,24.,3.));
#15971=CARTESIAN_POINT('Origin',(-39.,24.,2.));
#15972=CARTESIAN_POINT('',(-40.,24.,2.));
#15973=CARTESIAN_POINT('Origin',(-39.,24.,2.));
#15974=CARTESIAN_POINT('Origin',(-39.,24.,2.));
#15975=CARTESIAN_POINT('Origin',(39.,24.,1.));
#15976=CARTESIAN_POINT('',(40.,24.,1.));
#15977=CARTESIAN_POINT('',(39.,25.,1.));
#15978=CARTESIAN_POINT('Origin',(39.,24.,1.));
#15979=CARTESIAN_POINT('',(39.,24.,0.));
#15980=CARTESIAN_POINT('Origin',(39.,24.,1.));
#15981=CARTESIAN_POINT('Origin',(39.,24.,1.));
#15982=CARTESIAN_POINT('Origin',(39.,-24.,2.));
#15983=CARTESIAN_POINT('',(39.,-25.,2.));
#15984=CARTESIAN_POINT('',(39.,-24.,3.));
#15985=CARTESIAN_POINT('Origin',(39.,-24.,2.));
#15986=CARTESIAN_POINT('',(40.,-24.,2.));
#15987=CARTESIAN_POINT('Origin',(39.,-24.,2.));
#15988=CARTESIAN_POINT('Origin',(39.,-24.,2.));
#15989=CARTESIAN_POINT('Origin',(-39.,24.,1.));
#15990=CARTESIAN_POINT('',(-39.,24.,0.));
#15991=CARTESIAN_POINT('',(-39.,25.,1.));
#15992=CARTESIAN_POINT('Origin',(-39.,24.,1.));
#15993=CARTESIAN_POINT('',(-40.,24.,1.));
#15994=CARTESIAN_POINT('Origin',(-39.,24.,1.));
#15995=CARTESIAN_POINT('Origin',(-39.,24.,1.));
#15996=CARTESIAN_POINT('Origin',(-39.,-24.,2.));
#15997=CARTESIAN_POINT('',(-40.,-24.,2.));
#15998=CARTESIAN_POINT('',(-39.,-24.,3.));
#15999=CARTESIAN_POINT('Origin',(-39.,-24.,2.));
#16000=CARTESIAN_POINT('',(-39.,-25.,2.));
#16001=CARTESIAN_POINT('Origin',(-39.,-24.,2.));
#16002=CARTESIAN_POINT('Origin',(-39.,-24.,2.));
#16003=CARTESIAN_POINT('Origin',(39.,-24.,1.));
#16004=CARTESIAN_POINT('',(39.,-25.,1.));
#16005=CARTESIAN_POINT('',(40.,-24.,1.));
#16006=CARTESIAN_POINT('Origin',(39.,-24.,1.));
#16007=CARTESIAN_POINT('',(39.,-24.,0.));
#16008=CARTESIAN_POINT('Origin',(39.,-24.,1.));
#16009=CARTESIAN_POINT('Origin',(39.,-24.,1.));
#16010=CARTESIAN_POINT('Origin',(-39.,-24.,1.));
#16011=CARTESIAN_POINT('',(-40.,-24.,1.));
#16012=CARTESIAN_POINT('',(-39.,-25.,1.));
#16013=CARTESIAN_POINT('Origin',(-39.,-24.,1.));
#16014=CARTESIAN_POINT('',(-39.,-24.,0.));
#16015=CARTESIAN_POINT('Origin',(-39.,-24.,1.));
#16016=CARTESIAN_POINT('Origin',(-39.,-24.,1.));
#16017=CARTESIAN_POINT('Origin',(-39.,12.5,1.));
#16018=CARTESIAN_POINT('',(-40.,12.5,1.));
#16019=CARTESIAN_POINT('',(-39.,12.5,0.));
#16020=CARTESIAN_POINT('Origin',(-20.,-24.,1.));
#16021=CARTESIAN_POINT('',(-20.,-25.,1.));
#16022=CARTESIAN_POINT('',(-20.,-24.,0.));
#16023=CARTESIAN_POINT('Origin',(-39.,-24.,0.));
#16024=CARTESIAN_POINT('',(-40.,-24.,0.));
#16025=CARTESIAN_POINT('',(-39.,-25.,0.));
#16026=CARTESIAN_POINT('Origin',(39.,-12.5,1.));
#16027=CARTESIAN_POINT('',(40.,-12.5,1.));
#16028=CARTESIAN_POINT('',(39.,-12.5,0.));
#16029=CARTESIAN_POINT('Origin',(39.,-24.,0.));
#16030=CARTESIAN_POINT('',(39.,-25.,0.));
#16031=CARTESIAN_POINT('',(40.,-24.,0.));
#16032=CARTESIAN_POINT('Origin',(-20.,-24.,2.));
#16033=CARTESIAN_POINT('',(-20.,-24.,3.));
#16034=CARTESIAN_POINT('',(-20.,-25.,2.));
#16035=CARTESIAN_POINT('Origin',(-39.,12.5,2.));
#16036=CARTESIAN_POINT('',(-39.,12.5,3.));
#16037=CARTESIAN_POINT('',(-40.,12.5,2.));
#16038=CARTESIAN_POINT('Origin',(-39.,24.,0.));
#16039=CARTESIAN_POINT('',(-39.,25.,0.));
#16040=CARTESIAN_POINT('',(-40.,24.,0.));
#16041=CARTESIAN_POINT('Origin',(20.,24.,1.));
#16042=CARTESIAN_POINT('',(20.,25.,1.));
#16043=CARTESIAN_POINT('',(20.,24.,0.));
#16044=CARTESIAN_POINT('Origin',(39.,-12.5,2.));
#16045=CARTESIAN_POINT('',(39.,-12.5,3.));
#16046=CARTESIAN_POINT('',(40.,-12.5,2.));
#16047=CARTESIAN_POINT('Origin',(39.,24.,0.));
#16048=CARTESIAN_POINT('',(40.,24.,0.));
#16049=CARTESIAN_POINT('',(39.,25.,0.));
#16050=CARTESIAN_POINT('Origin',(20.,24.,2.));
#16051=CARTESIAN_POINT('',(20.,24.,3.));
#16052=CARTESIAN_POINT('',(20.,25.,2.));
#16053=CARTESIAN_POINT('Origin',(-40.,25.,0.));
#16054=CARTESIAN_POINT('Origin',(0.,0.,0.));
#16055=CARTESIAN_POINT('',(-21.,-15.,0.));
#16056=CARTESIAN_POINT('',(21.,-15.,0.));
#16057=CARTESIAN_POINT('',(10.5,-15.,0.));
#16058=CARTESIAN_POINT('',(21.,15.,0.));
#16059=CARTESIAN_POINT('',(21.,7.5,0.));
#16060=CARTESIAN_POINT('',(-21.,15.,0.));
#16061=CARTESIAN_POINT('',(-10.5,15.,0.));
#16062=CARTESIAN_POINT('',(-21.,-7.5,0.));
#16063=CARTESIAN_POINT('',(24.5,4.28626379701574E-16,0.));
#16064=CARTESIAN_POINT('Origin',(28.,0.,0.));
#16065=CARTESIAN_POINT('',(-31.5,4.28626379701574E-16,0.));
#16066=CARTESIAN_POINT('Origin',(-28.,0.,0.));
#16067=CARTESIAN_POINT('Origin',(-40.,-25.,0.));
#16068=CARTESIAN_POINT('Origin',(40.,-25.,0.));
#16069=CARTESIAN_POINT('Origin',(0.,0.,3.));
#16070=CARTESIAN_POINT('',(21.,-15.,3.));
#16071=CARTESIAN_POINT('',(-21.,-15.,3.));
#16072=CARTESIAN_POINT('',(10.5,-15.,3.));
#16073=CARTESIAN_POINT('',(-21.,15.,3.));
#16074=CARTESIAN_POINT('',(-21.,-7.5,3.));
#16075=CARTESIAN_POINT('',(21.,15.,3.));
#16076=CARTESIAN_POINT('',(-10.5,15.,3.));
#16077=CARTESIAN_POINT('',(21.,7.5,3.));
#16078=CARTESIAN_POINT('',(24.5,4.28626379701574E-16,3.));
#16079=CARTESIAN_POINT('Origin',(28.,0.,3.));
#16080=CARTESIAN_POINT('',(-31.5,4.28626379701574E-16,3.));
#16081=CARTESIAN_POINT('Origin',(-28.,0.,3.));
#16082=CARTESIAN_POINT('Origin',(40.,25.,0.));
#16083=CARTESIAN_POINT('Origin',(-28.,0.,1.5));
#16084=CARTESIAN_POINT('',(-31.5,4.28626379701574E-16,1.5));
#16085=CARTESIAN_POINT('Origin',(28.,0.,1.5));
#16086=CARTESIAN_POINT('',(24.5,4.28626379701574E-16,1.5));
#16087=CARTESIAN_POINT('Origin',(21.,-15.,3.));
#16088=CARTESIAN_POINT('',(21.,-15.,3.));
#16089=CARTESIAN_POINT('',(-21.,-15.,3.));
#16090=CARTESIAN_POINT('Origin',(21.,15.,3.));
#16091=CARTESIAN_POINT('',(21.,15.,3.));
#16092=CARTESIAN_POINT('Origin',(-21.,15.,3.));
#16093=CARTESIAN_POINT('',(-21.,15.,3.));
#16094=CARTESIAN_POINT('Origin',(-21.,-15.,3.));
#21859=UNCERTAINTY_MEASURE_WITH_UNIT(LENGTH_MEASURE(0.01),#21881,
'DISTANCE_ACCURACY_VALUE',
'Maximum model space distance between geometric entities at asserted c
onnectivities');
#21868=UNCERTAINTY_MEASURE_WITH_UNIT(LENGTH_MEASURE(0.01),#21881,
'DISTANCE_ACCURACY_VALUE',
'Maximum model space distance between geometric entities at asserted c
onnectivities');
#21871=(
GEOMETRIC_REPRESENTATION_CONTEXT(3)
GLOBAL_UNCERTAINTY_ASSIGNED_CONTEXT((#21859))
GLOBAL_UNIT_ASSIGNED_CONTEXT((#21881,#21883,#21884))
REPRESENTATION_CONTEXT('','3D')
);
#21880=(
GEOMETRIC_REPRESENTATION_CONTEXT(3)
GLOBAL_UNCERTAINTY_ASSIGNED_CONTEXT((#21868))
GLOBAL_UNIT_ASSIGNED_CONTEXT((#21881,#21883,#21884))
REPRESENTATION_CONTEXT('','3D')
);
#21881=(
LENGTH_UNIT()
NAMED_UNIT(*)
SI_UNIT(.MILLI.,.METRE.)
);
#21883=(
NAMED_UNIT(*)
PLANE_ANGLE_UNIT()
SI_UNIT($,.RADIAN.)
);
#21884=(
NAMED_UNIT(*)
SI_UNIT($,.STERADIAN.)
SOLID_ANGLE_UNIT()
);
#21887=SHAPE_DEFINITION_REPRESENTATION(#21898,#21926);
#21898=PRODUCT_DEFINITION_SHAPE('',$,#21938);
#21926=SHAPE_REPRESENTATION('',(#6693),#21871);
#21935=PRODUCT_DEFINITION_CONTEXT('part definition',#21970,'design');
#21938=PRODUCT_DEFINITION('Panel plate','Panel plate',#21949,#21935);
#21949=PRODUCT_DEFINITION_FORMATION('',$,#21974);
#21970=APPLICATION_CONTEXT(
'Core Data for Automotive Mechanical Design Process');
#21971=PRODUCT_CONTEXT('part definition',#21970,'mechanical');
#21974=PRODUCT('Panel plate','Panel plate',$,(#21971));
#21985=PRESENTATION_STYLE_ASSIGNMENT((#21991));
#21991=SURFACE_STYLE_USAGE(.BOTH.,#21997);
#21997=SURFACE_SIDE_STYLE('',(#22003));
#22003=SURFACE_STYLE_FILL_AREA(#22009);
#22009=FILL_AREA_STYLE('Gray',(#22015));
#22015=FILL_AREA_STYLE_COLOUR('Gray',#22021);
#22021=COLOUR_RGB('Gray',0.407843137254902,0.447058823529412,0.498039215686275);
ENDSEC;
END-ISO-10303-21;
